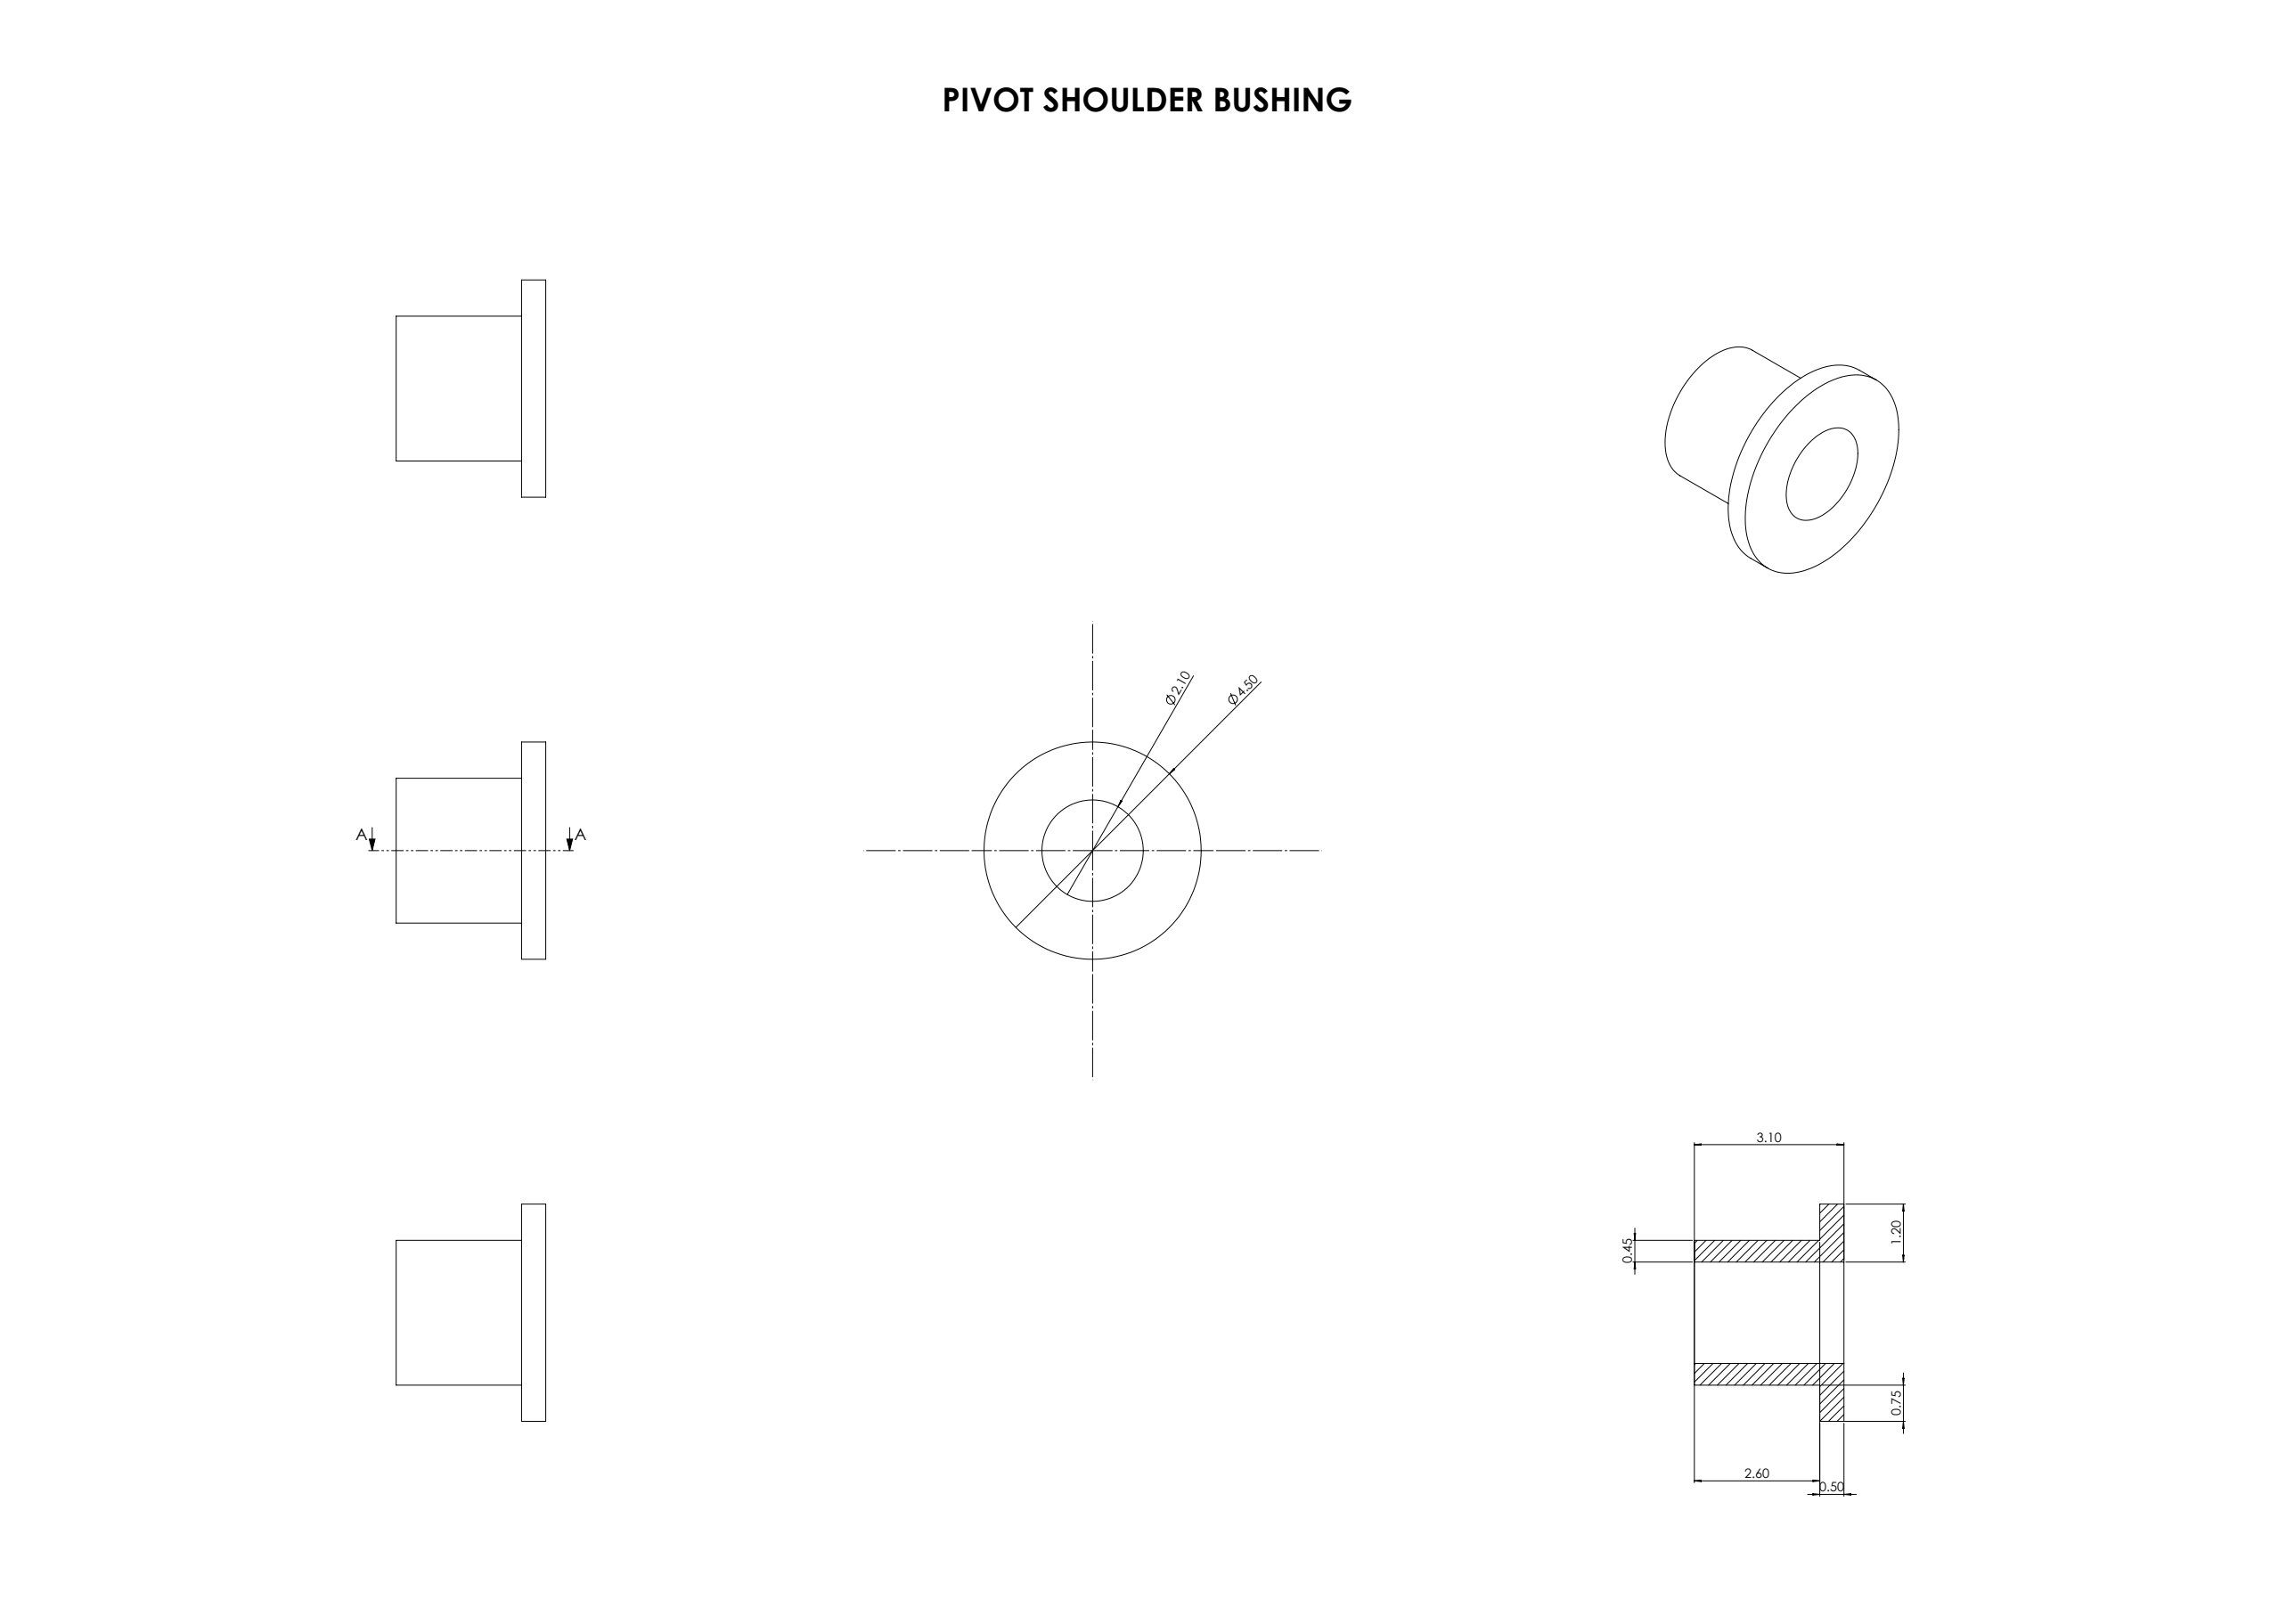
ISO-10303-21;
HEADER;
/* Generated by software containing ST-Developer
 * from STEP Tools, Inc. (www.steptools.com) 
 */

FILE_DESCRIPTION(
/* description */ (''),
/* implementation_level */ '2;1');

FILE_NAME(
/* name */ '09_Pivot_Shoulder_Bushing.step',
/* time_stamp */ '2026-10-25T01:35:35-07:00',
/* author */ (''),
/* organization */ (''),
/* preprocessor_version */ 'ST-DEVELOPER v20.2',
/* originating_system */ 'Autodesk Translation Framework v15.15.0.0',
/* authorisation */ '');

FILE_SCHEMA (('AUTOMOTIVE_DESIGN { 1 0 10303 214 3 1 1 }'));
ENDSEC;

DATA;
#10=MECHANICAL_DESIGN_GEOMETRIC_PRESENTATION_REPRESENTATION('',(#269),#11430);
#245=SHAPE_REPRESENTATION_RELATIONSHIP('SRR','None',#11488,#257);
#257=ADVANCED_BREP_SHAPE_REPRESENTATION('',(#281),#11427);
#269=STYLED_ITEM('',(#11623),#281);
#281=MANIFOLD_SOLID_BREP('Body1',#4470);
#316=FACE_BOUND('',#1034,.T.);
#317=FACE_BOUND('',#1037,.T.);
#318=FACE_BOUND('',#1040,.T.);
#409=PLANE('',#4981);
#410=PLANE('',#4985);
#411=PLANE('',#4989);
#494=CYLINDRICAL_SURFACE('',#4978,1.05);
#495=CYLINDRICAL_SURFACE('',#4983,1.5);
#496=CYLINDRICAL_SURFACE('',#4987,2.25);
#732=FACE_OUTER_BOUND('',#1032,.T.);
#733=FACE_OUTER_BOUND('',#1033,.T.);
#734=FACE_OUTER_BOUND('',#1035,.T.);
#735=FACE_OUTER_BOUND('',#1036,.T.);
#736=FACE_OUTER_BOUND('',#1038,.T.);
#737=FACE_OUTER_BOUND('',#1039,.T.);
#1032=EDGE_LOOP('',(#3827,#3828,#3829,#3830));
#1033=EDGE_LOOP('',(#3831));
#1034=EDGE_LOOP('',(#3832));
#1035=EDGE_LOOP('',(#3833,#3834,#3835,#3836));
#1036=EDGE_LOOP('',(#3837));
#1037=EDGE_LOOP('',(#3838));
#1038=EDGE_LOOP('',(#3839,#3840,#3841,#3842));
#1039=EDGE_LOOP('',(#3843));
#1040=EDGE_LOOP('',(#3844));
#1319=LINE('',#9375,#1609);
#1320=LINE('',#9383,#1610);
#1321=LINE('',#9390,#1611);
#1609=VECTOR('',#6049,1.05);
#1610=VECTOR('',#6060,1.5);
#1611=VECTOR('',#6069,2.25);
#1840=CIRCLE('',#4979,1.05);
#1841=CIRCLE('',#4980,1.05);
#1842=CIRCLE('',#4982,1.5);
#1843=CIRCLE('',#4984,1.5);
#1844=CIRCLE('',#4986,2.25);
#1845=CIRCLE('',#4988,2.25);
#2159=VERTEX_POINT('',#9372);
#2160=VERTEX_POINT('',#9374);
#2161=VERTEX_POINT('',#9378);
#2162=VERTEX_POINT('',#9381);
#2163=VERTEX_POINT('',#9385);
#2164=VERTEX_POINT('',#9388);
#2731=EDGE_CURVE('',#2159,#2159,#1840,.T.);
#2732=EDGE_CURVE('',#2159,#2160,#1319,.T.);
#2733=EDGE_CURVE('',#2160,#2160,#1841,.T.);
#2734=EDGE_CURVE('',#2161,#2161,#1842,.T.);
#2735=EDGE_CURVE('',#2162,#2162,#1843,.T.);
#2736=EDGE_CURVE('',#2162,#2161,#1320,.T.);
#2737=EDGE_CURVE('',#2163,#2163,#1844,.T.);
#2738=EDGE_CURVE('',#2164,#2164,#1845,.T.);
#2739=EDGE_CURVE('',#2164,#2163,#1321,.T.);
#3827=ORIENTED_EDGE('',*,*,#2731,.T.);
#3828=ORIENTED_EDGE('',*,*,#2732,.T.);
#3829=ORIENTED_EDGE('',*,*,#2733,.F.);
#3830=ORIENTED_EDGE('',*,*,#2732,.F.);
#3831=ORIENTED_EDGE('',*,*,#2734,.F.);
#3832=ORIENTED_EDGE('',*,*,#2733,.T.);
#3833=ORIENTED_EDGE('',*,*,#2735,.F.);
#3834=ORIENTED_EDGE('',*,*,#2736,.T.);
#3835=ORIENTED_EDGE('',*,*,#2734,.T.);
#3836=ORIENTED_EDGE('',*,*,#2736,.F.);
#3837=ORIENTED_EDGE('',*,*,#2737,.F.);
#3838=ORIENTED_EDGE('',*,*,#2735,.T.);
#3839=ORIENTED_EDGE('',*,*,#2738,.F.);
#3840=ORIENTED_EDGE('',*,*,#2739,.T.);
#3841=ORIENTED_EDGE('',*,*,#2737,.T.);
#3842=ORIENTED_EDGE('',*,*,#2739,.F.);
#3843=ORIENTED_EDGE('',*,*,#2738,.T.);
#3844=ORIENTED_EDGE('',*,*,#2731,.F.);
#4399=ADVANCED_FACE('',(#732),#494,.F.);
#4400=ADVANCED_FACE('',(#733,#316),#409,.T.);
#4401=ADVANCED_FACE('',(#734),#495,.T.);
#4402=ADVANCED_FACE('',(#735,#317),#410,.T.);
#4403=ADVANCED_FACE('',(#736),#496,.T.);
#4404=ADVANCED_FACE('',(#737,#318),#411,.T.);
#4470=CLOSED_SHELL('',(#4399,#4400,#4401,#4402,#4403,#4404));
#4977=AXIS2_PLACEMENT_3D('',#9370,#6043,#6044);
#4978=AXIS2_PLACEMENT_3D('',#9371,#6045,#6046);
#4979=AXIS2_PLACEMENT_3D('',#9373,#6047,#6048);
#4980=AXIS2_PLACEMENT_3D('',#9376,#6050,#6051);
#4981=AXIS2_PLACEMENT_3D('',#9377,#6052,#6053);
#4982=AXIS2_PLACEMENT_3D('',#9379,#6054,#6055);
#4983=AXIS2_PLACEMENT_3D('',#9380,#6056,#6057);
#4984=AXIS2_PLACEMENT_3D('',#9382,#6058,#6059);
#4985=AXIS2_PLACEMENT_3D('',#9384,#6061,#6062);
#4986=AXIS2_PLACEMENT_3D('',#9386,#6063,#6064);
#4987=AXIS2_PLACEMENT_3D('',#9387,#6065,#6066);
#4988=AXIS2_PLACEMENT_3D('',#9389,#6067,#6068);
#4989=AXIS2_PLACEMENT_3D('',#9391,#6070,#6071);
#6043=DIRECTION('axis',(0.,0.,1.));
#6044=DIRECTION('refdir',(1.,0.,0.));
#6045=DIRECTION('center_axis',(1.,0.,0.));
#6046=DIRECTION('ref_axis',(0.,1.,0.));
#6047=DIRECTION('center_axis',(1.,0.,0.));
#6048=DIRECTION('ref_axis',(0.,0.,-1.));
#6049=DIRECTION('',(-1.,0.,0.));
#6050=DIRECTION('center_axis',(1.,0.,0.));
#6051=DIRECTION('ref_axis',(0.,0.,-1.));
#6052=DIRECTION('center_axis',(-1.,0.,0.));
#6053=DIRECTION('ref_axis',(0.,0.,1.));
#6054=DIRECTION('center_axis',(1.,0.,0.));
#6055=DIRECTION('ref_axis',(0.,0.,-1.));
#6056=DIRECTION('center_axis',(1.,0.,0.));
#6057=DIRECTION('ref_axis',(0.,1.,0.));
#6058=DIRECTION('center_axis',(1.,0.,0.));
#6059=DIRECTION('ref_axis',(0.,0.,-1.));
#6060=DIRECTION('',(-1.,0.,0.));
#6061=DIRECTION('center_axis',(-1.,0.,0.));
#6062=DIRECTION('ref_axis',(0.,0.,1.));
#6063=DIRECTION('center_axis',(1.,0.,0.));
#6064=DIRECTION('ref_axis',(0.,0.,-1.));
#6065=DIRECTION('center_axis',(1.,0.,0.));
#6066=DIRECTION('ref_axis',(0.,1.,0.));
#6067=DIRECTION('center_axis',(1.,0.,0.));
#6068=DIRECTION('ref_axis',(0.,0.,-1.));
#6069=DIRECTION('',(-1.,0.,0.));
#6070=DIRECTION('center_axis',(1.,0.,0.));
#6071=DIRECTION('ref_axis',(0.,0.,-1.));
#9370=CARTESIAN_POINT('',(0.,0.,0.));
#9371=CARTESIAN_POINT('Origin',(1.55,0.,0.));
#9372=CARTESIAN_POINT('',(3.1,-1.05,-1.28587913910472E-16));
#9373=CARTESIAN_POINT('Origin',(3.1,0.,0.));
#9374=CARTESIAN_POINT('',(0.,-1.05,-1.28587913910472E-16));
#9375=CARTESIAN_POINT('',(1.55,-1.05,-1.28587913910472E-16));
#9376=CARTESIAN_POINT('Origin',(0.,0.,0.));
#9377=CARTESIAN_POINT('Origin',(0.,1.5,0.));
#9378=CARTESIAN_POINT('',(0.,-1.5,-1.83697019872103E-16));
#9379=CARTESIAN_POINT('Origin',(0.,0.,0.));
#9380=CARTESIAN_POINT('Origin',(1.3,0.,0.));
#9381=CARTESIAN_POINT('',(2.6,-1.5,-1.83697019872103E-16));
#9382=CARTESIAN_POINT('Origin',(2.6,0.,0.));
#9383=CARTESIAN_POINT('',(1.3,-1.5,-1.83697019872103E-16));
#9384=CARTESIAN_POINT('Origin',(2.6,2.25,0.));
#9385=CARTESIAN_POINT('',(2.6,-2.25,-2.75545529808154E-16));
#9386=CARTESIAN_POINT('Origin',(2.6,0.,0.));
#9387=CARTESIAN_POINT('Origin',(2.85,0.,0.));
#9388=CARTESIAN_POINT('',(3.1,-2.25,-2.75545529808154E-16));
#9389=CARTESIAN_POINT('Origin',(3.1,0.,0.));
#9390=CARTESIAN_POINT('',(2.85,-2.25,-2.75545529808154E-16));
#9391=CARTESIAN_POINT('Origin',(3.1,1.05,0.));
#11413=UNCERTAINTY_MEASURE_WITH_UNIT(LENGTH_MEASURE(0.01),#11431,
'DISTANCE_ACCURACY_VALUE',
'Maximum model space distance between geometric entities at asserted c
onnectivities');
#11416=UNCERTAINTY_MEASURE_WITH_UNIT(LENGTH_MEASURE(0.01),#11431,
'DISTANCE_ACCURACY_VALUE',
'Maximum model space distance between geometric entities at asserted c
onnectivities');
#11427=(
GEOMETRIC_REPRESENTATION_CONTEXT(3)
GLOBAL_UNCERTAINTY_ASSIGNED_CONTEXT((#11413))
GLOBAL_UNIT_ASSIGNED_CONTEXT((#11431,#11433,#11434))
REPRESENTATION_CONTEXT('','3D')
);
#11430=(
GEOMETRIC_REPRESENTATION_CONTEXT(3)
GLOBAL_UNCERTAINTY_ASSIGNED_CONTEXT((#11416))
GLOBAL_UNIT_ASSIGNED_CONTEXT((#11431,#11433,#11434))
REPRESENTATION_CONTEXT('','3D')
);
#11431=(
LENGTH_UNIT()
NAMED_UNIT(*)
SI_UNIT(.MILLI.,.METRE.)
);
#11433=(
NAMED_UNIT(*)
PLANE_ANGLE_UNIT()
SI_UNIT($,.RADIAN.)
);
#11434=(
NAMED_UNIT(*)
SI_UNIT($,.STERADIAN.)
SOLID_ANGLE_UNIT()
);
#11445=SHAPE_DEFINITION_REPRESENTATION(#11458,#11488);
#11458=PRODUCT_DEFINITION_SHAPE('',$,#11502);
#11488=SHAPE_REPRESENTATION('',(#4977),#11427);
#11491=PRODUCT_DEFINITION_CONTEXT('part definition',#11532,'design');
#11502=PRODUCT_DEFINITION('2026-10-25-00-55-40-297',
'09_Pivot_Shoulder_Bushing',#11515,#11491);
#11515=PRODUCT_DEFINITION_FORMATION('',$,#11544);
#11532=APPLICATION_CONTEXT(
'Core Data for Automotive Mechanical Design Process');
#11533=PRODUCT_CONTEXT('part definition',#11532,'mechanical');
#11544=PRODUCT('2026-10-25-00-55-40-297','09_Pivot_Shoulder_Bushing',$,
(#11533));
#11617=COLOUR_RGB('Off White',0.89,0.88,0.83);
#11618=FILL_AREA_STYLE_COLOUR('',#11617);
#11619=FILL_AREA_STYLE('',(#11618));
#11620=SURFACE_STYLE_FILL_AREA(#11619);
#11621=SURFACE_SIDE_STYLE('',(#11620));
#11622=SURFACE_STYLE_USAGE(.BOTH.,#11621);
#11623=PRESENTATION_STYLE_ASSIGNMENT((#11622));
ENDSEC;
END-ISO-10303-21;
